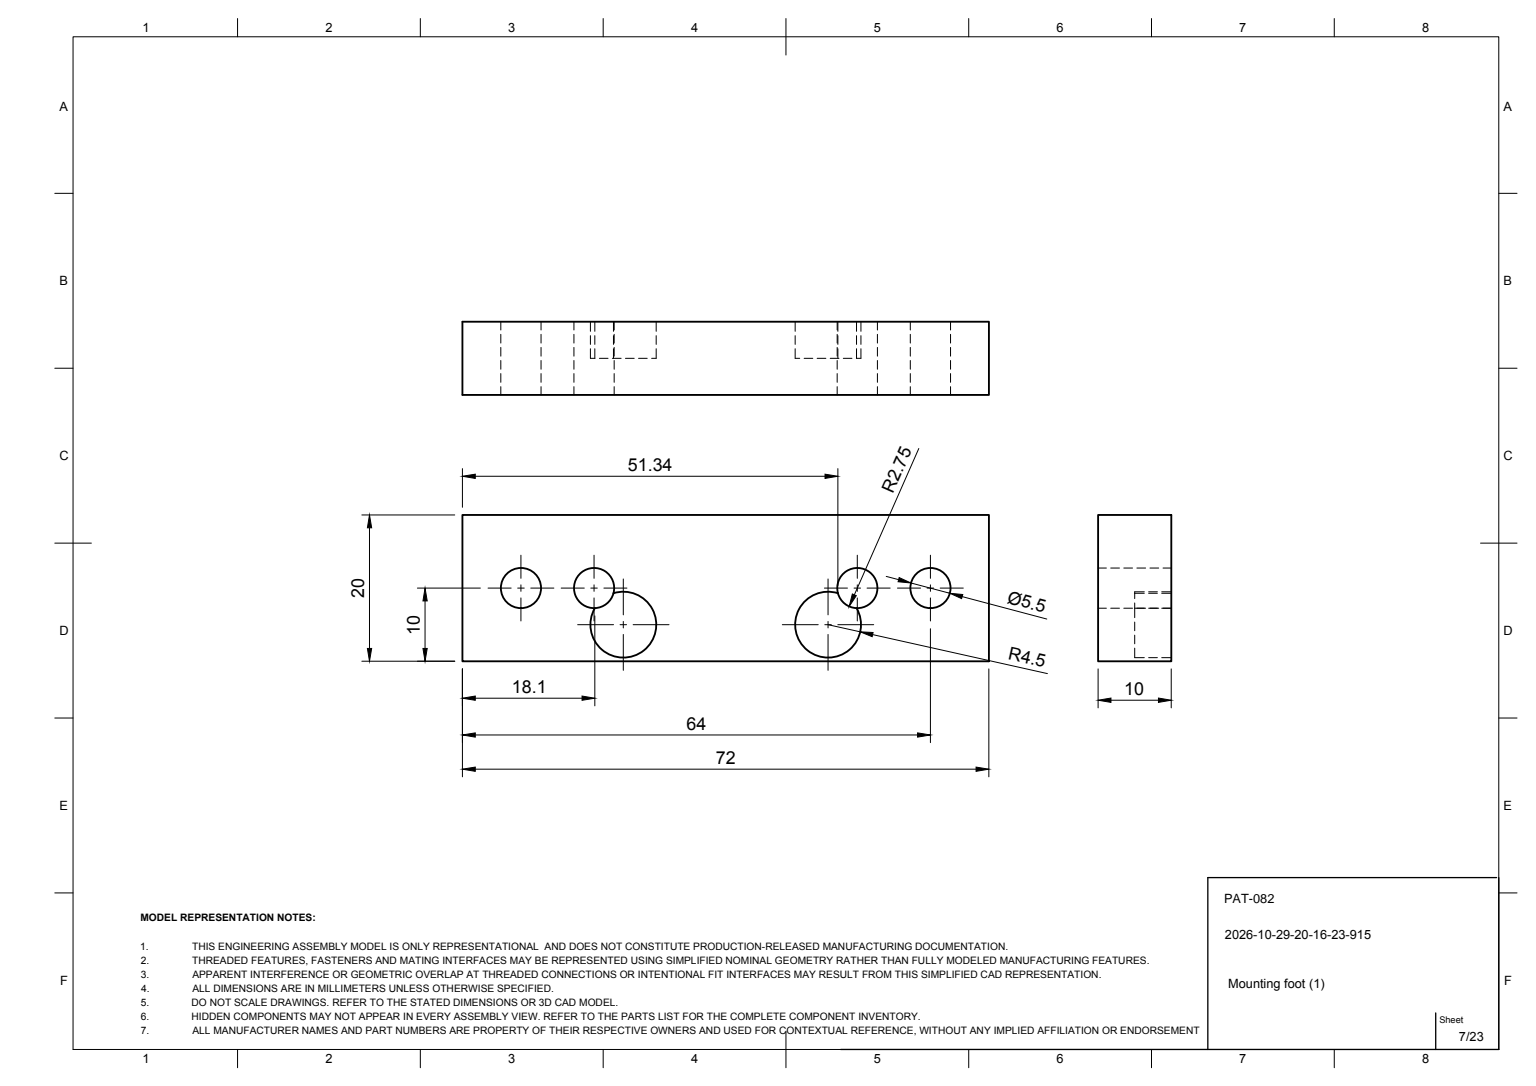
ISO-10303-21;
HEADER;
/* Generated by software containing ST-Developer
 * from STEP Tools, Inc. (www.steptools.com) 
 */

FILE_DESCRIPTION(
/* description */ ('PAT-082'),
/* implementation_level */ '2;1');

FILE_NAME(
/* name */ 'Mounting foot (1).step',
/* time_stamp */ '2026-10-29T20:16:13-07:00',
/* author */ (''),
/* organization */ (''),
/* preprocessor_version */ 'ST-DEVELOPER v20.2',
/* originating_system */ 'Autodesk Translation Framework v15.17.0.0',
/* authorisation */ '');

FILE_SCHEMA (('AUTOMOTIVE_DESIGN { 1 0 10303 214 3 1 1 }'));
ENDSEC;

DATA;
#10=MECHANICAL_DESIGN_GEOMETRIC_PRESENTATION_REPRESENTATION('',(#245),#8266);
#201=SHAPE_REPRESENTATION_RELATIONSHIP('SRR','None',#8363,#223);
#223=ADVANCED_BREP_SHAPE_REPRESENTATION('',(#267),#8247);
#245=STYLED_ITEM('',(#8530),#267);
#267=MANIFOLD_SOLID_BREP('Body1',#4585);
#302=FACE_BOUND('',#919,.T.);
#303=FACE_BOUND('',#920,.T.);
#304=FACE_BOUND('',#921,.T.);
#305=FACE_BOUND('',#922,.T.);
#306=FACE_BOUND('',#924,.T.);
#307=FACE_BOUND('',#925,.T.);
#308=FACE_BOUND('',#926,.T.);
#309=FACE_BOUND('',#927,.T.);
#435=PLANE('',#4931);
#436=PLANE('',#4936);
#437=PLANE('',#4955);
#438=PLANE('',#4956);
#439=PLANE('',#4957);
#440=PLANE('',#4958);
#441=PLANE('',#4959);
#442=PLANE('',#4960);
#616=FACE_OUTER_BOUND('',#906,.T.);
#617=FACE_OUTER_BOUND('',#907,.T.);
#618=FACE_OUTER_BOUND('',#908,.T.);
#619=FACE_OUTER_BOUND('',#909,.T.);
#620=FACE_OUTER_BOUND('',#910,.T.);
#621=FACE_OUTER_BOUND('',#911,.T.);
#622=FACE_OUTER_BOUND('',#912,.T.);
#623=FACE_OUTER_BOUND('',#913,.T.);
#624=FACE_OUTER_BOUND('',#914,.T.);
#625=FACE_OUTER_BOUND('',#915,.T.);
#626=FACE_OUTER_BOUND('',#916,.T.);
#627=FACE_OUTER_BOUND('',#917,.T.);
#628=FACE_OUTER_BOUND('',#918,.T.);
#629=FACE_OUTER_BOUND('',#923,.T.);
#906=EDGE_LOOP('',(#3278,#3279));
#907=EDGE_LOOP('',(#3280,#3281,#3282,#3283));
#908=EDGE_LOOP('',(#3284,#3285));
#909=EDGE_LOOP('',(#3286,#3287,#3288,#3289));
#910=EDGE_LOOP('',(#3290,#3291,#3292,#3293,#3294,#3295,#3296,#3297));
#911=EDGE_LOOP('',(#3298,#3299,#3300,#3301,#3302,#3303,#3304,#3305));
#912=EDGE_LOOP('',(#3306,#3307,#3308,#3309));
#913=EDGE_LOOP('',(#3310,#3311,#3312,#3313));
#914=EDGE_LOOP('',(#3314,#3315,#3316,#3317));
#915=EDGE_LOOP('',(#3318,#3319,#3320,#3321));
#916=EDGE_LOOP('',(#3322,#3323,#3324,#3325));
#917=EDGE_LOOP('',(#3326,#3327,#3328,#3329));
#918=EDGE_LOOP('',(#3330,#3331,#3332,#3333));
#919=EDGE_LOOP('',(#3334,#3335,#3336));
#920=EDGE_LOOP('',(#3337,#3338,#3339));
#921=EDGE_LOOP('',(#3340));
#922=EDGE_LOOP('',(#3341));
#923=EDGE_LOOP('',(#3342,#3343,#3344,#3345));
#924=EDGE_LOOP('',(#3346));
#925=EDGE_LOOP('',(#3347));
#926=EDGE_LOOP('',(#3348));
#927=EDGE_LOOP('',(#3349));
#1299=LINE('',#7020,#1654);
#1300=LINE('',#7023,#1655);
#1301=LINE('',#7031,#1656);
#1302=LINE('',#7034,#1657);
#1303=LINE('',#7039,#1658);
#1304=LINE('',#7046,#1659);
#1305=LINE('',#7053,#1660);
#1306=LINE('',#7059,#1661);
#1307=LINE('',#7064,#1662);
#1308=LINE('',#7066,#1663);
#1309=LINE('',#7068,#1664);
#1310=LINE('',#7069,#1665);
#1311=LINE('',#7072,#1666);
#1312=LINE('',#7074,#1667);
#1313=LINE('',#7075,#1668);
#1314=LINE('',#7078,#1669);
#1315=LINE('',#7080,#1670);
#1316=LINE('',#7081,#1671);
#1317=LINE('',#7083,#1672);
#1318=LINE('',#7084,#1673);
#1654=VECTOR('',#5618,1.);
#1655=VECTOR('',#5621,1.);
#1656=VECTOR('',#5630,1.);
#1657=VECTOR('',#5633,1.);
#1658=VECTOR('',#5638,0.275);
#1659=VECTOR('',#5647,0.275);
#1660=VECTOR('',#5656,0.275);
#1661=VECTOR('',#5663,0.275);
#1662=VECTOR('',#5668,1.);
#1663=VECTOR('',#5669,1.);
#1664=VECTOR('',#5670,1.);
#1665=VECTOR('',#5671,1.);
#1666=VECTOR('',#5674,1.);
#1667=VECTOR('',#5675,1.);
#1668=VECTOR('',#5676,1.);
#1669=VECTOR('',#5679,1.);
#1670=VECTOR('',#5680,1.);
#1671=VECTOR('',#5681,1.);
#1672=VECTOR('',#5684,1.);
#1673=VECTOR('',#5685,1.);
#1977=CIRCLE('',#4932,0.275);
#1978=CIRCLE('',#4933,0.45);
#1979=CIRCLE('',#4935,0.45);
#1980=CIRCLE('',#4937,0.275);
#1981=CIRCLE('',#4938,0.45);
#1982=CIRCLE('',#4940,0.45);
#1983=CIRCLE('',#4942,0.275);
#1984=CIRCLE('',#4943,0.275);
#1985=CIRCLE('',#4944,0.275);
#1986=CIRCLE('',#4946,0.275);
#1987=CIRCLE('',#4947,0.275);
#1988=CIRCLE('',#4948,0.275);
#1989=CIRCLE('',#4950,0.275);
#1990=CIRCLE('',#4951,0.275);
#1991=CIRCLE('',#4953,0.275);
#1992=CIRCLE('',#4954,0.275);
#2209=VERTEX_POINT('',#7014);
#2210=VERTEX_POINT('',#7015);
#2211=VERTEX_POINT('',#7019);
#2212=VERTEX_POINT('',#7021);
#2213=VERTEX_POINT('',#7025);
#2214=VERTEX_POINT('',#7026);
#2215=VERTEX_POINT('',#7030);
#2216=VERTEX_POINT('',#7032);
#2217=VERTEX_POINT('',#7036);
#2218=VERTEX_POINT('',#7038);
#2219=VERTEX_POINT('',#7043);
#2220=VERTEX_POINT('',#7045);
#2221=VERTEX_POINT('',#7050);
#2222=VERTEX_POINT('',#7052);
#2223=VERTEX_POINT('',#7056);
#2224=VERTEX_POINT('',#7058);
#2225=VERTEX_POINT('',#7062);
#2226=VERTEX_POINT('',#7063);
#2227=VERTEX_POINT('',#7065);
#2228=VERTEX_POINT('',#7067);
#2229=VERTEX_POINT('',#7071);
#2230=VERTEX_POINT('',#7073);
#2231=VERTEX_POINT('',#7077);
#2232=VERTEX_POINT('',#7079);
#2615=EDGE_CURVE('',#2209,#2210,#1977,.T.);
#2616=EDGE_CURVE('',#2209,#2210,#1978,.T.);
#2617=EDGE_CURVE('',#2211,#2209,#1299,.T.);
#2618=EDGE_CURVE('',#2212,#2211,#1979,.T.);
#2619=EDGE_CURVE('',#2210,#2212,#1300,.T.);
#2620=EDGE_CURVE('',#2213,#2214,#1980,.T.);
#2621=EDGE_CURVE('',#2213,#2214,#1981,.T.);
#2622=EDGE_CURVE('',#2215,#2213,#1301,.T.);
#2623=EDGE_CURVE('',#2216,#2215,#1982,.T.);
#2624=EDGE_CURVE('',#2214,#2216,#1302,.T.);
#2625=EDGE_CURVE('',#2217,#2217,#1983,.T.);
#2626=EDGE_CURVE('',#2217,#2218,#1303,.T.);
#2627=EDGE_CURVE('',#2211,#2218,#1984,.T.);
#2628=EDGE_CURVE('',#2218,#2212,#1985,.T.);
#2629=EDGE_CURVE('',#2219,#2219,#1986,.T.);
#2630=EDGE_CURVE('',#2219,#2220,#1304,.T.);
#2631=EDGE_CURVE('',#2215,#2220,#1987,.T.);
#2632=EDGE_CURVE('',#2220,#2216,#1988,.T.);
#2633=EDGE_CURVE('',#2221,#2221,#1989,.T.);
#2634=EDGE_CURVE('',#2221,#2222,#1305,.T.);
#2635=EDGE_CURVE('',#2222,#2222,#1990,.T.);
#2636=EDGE_CURVE('',#2223,#2223,#1991,.T.);
#2637=EDGE_CURVE('',#2223,#2224,#1306,.T.);
#2638=EDGE_CURVE('',#2224,#2224,#1992,.T.);
#2639=EDGE_CURVE('',#2225,#2226,#1307,.T.);
#2640=EDGE_CURVE('',#2226,#2227,#1308,.T.);
#2641=EDGE_CURVE('',#2228,#2227,#1309,.T.);
#2642=EDGE_CURVE('',#2225,#2228,#1310,.T.);
#2643=EDGE_CURVE('',#2229,#2225,#1311,.T.);
#2644=EDGE_CURVE('',#2230,#2228,#1312,.T.);
#2645=EDGE_CURVE('',#2229,#2230,#1313,.T.);
#2646=EDGE_CURVE('',#2231,#2229,#1314,.T.);
#2647=EDGE_CURVE('',#2232,#2230,#1315,.T.);
#2648=EDGE_CURVE('',#2231,#2232,#1316,.T.);
#2649=EDGE_CURVE('',#2226,#2231,#1317,.T.);
#2650=EDGE_CURVE('',#2227,#2232,#1318,.T.);
#3278=ORIENTED_EDGE('',*,*,#2615,.F.);
#3279=ORIENTED_EDGE('',*,*,#2616,.T.);
#3280=ORIENTED_EDGE('',*,*,#2617,.F.);
#3281=ORIENTED_EDGE('',*,*,#2618,.F.);
#3282=ORIENTED_EDGE('',*,*,#2619,.F.);
#3283=ORIENTED_EDGE('',*,*,#2616,.F.);
#3284=ORIENTED_EDGE('',*,*,#2620,.F.);
#3285=ORIENTED_EDGE('',*,*,#2621,.T.);
#3286=ORIENTED_EDGE('',*,*,#2622,.F.);
#3287=ORIENTED_EDGE('',*,*,#2623,.F.);
#3288=ORIENTED_EDGE('',*,*,#2624,.F.);
#3289=ORIENTED_EDGE('',*,*,#2621,.F.);
#3290=ORIENTED_EDGE('',*,*,#2625,.F.);
#3291=ORIENTED_EDGE('',*,*,#2626,.T.);
#3292=ORIENTED_EDGE('',*,*,#2627,.F.);
#3293=ORIENTED_EDGE('',*,*,#2617,.T.);
#3294=ORIENTED_EDGE('',*,*,#2615,.T.);
#3295=ORIENTED_EDGE('',*,*,#2619,.T.);
#3296=ORIENTED_EDGE('',*,*,#2628,.F.);
#3297=ORIENTED_EDGE('',*,*,#2626,.F.);
#3298=ORIENTED_EDGE('',*,*,#2629,.F.);
#3299=ORIENTED_EDGE('',*,*,#2630,.T.);
#3300=ORIENTED_EDGE('',*,*,#2631,.F.);
#3301=ORIENTED_EDGE('',*,*,#2622,.T.);
#3302=ORIENTED_EDGE('',*,*,#2620,.T.);
#3303=ORIENTED_EDGE('',*,*,#2624,.T.);
#3304=ORIENTED_EDGE('',*,*,#2632,.F.);
#3305=ORIENTED_EDGE('',*,*,#2630,.F.);
#3306=ORIENTED_EDGE('',*,*,#2633,.F.);
#3307=ORIENTED_EDGE('',*,*,#2634,.T.);
#3308=ORIENTED_EDGE('',*,*,#2635,.F.);
#3309=ORIENTED_EDGE('',*,*,#2634,.F.);
#3310=ORIENTED_EDGE('',*,*,#2636,.F.);
#3311=ORIENTED_EDGE('',*,*,#2637,.T.);
#3312=ORIENTED_EDGE('',*,*,#2638,.F.);
#3313=ORIENTED_EDGE('',*,*,#2637,.F.);
#3314=ORIENTED_EDGE('',*,*,#2639,.T.);
#3315=ORIENTED_EDGE('',*,*,#2640,.T.);
#3316=ORIENTED_EDGE('',*,*,#2641,.F.);
#3317=ORIENTED_EDGE('',*,*,#2642,.F.);
#3318=ORIENTED_EDGE('',*,*,#2643,.T.);
#3319=ORIENTED_EDGE('',*,*,#2642,.T.);
#3320=ORIENTED_EDGE('',*,*,#2644,.F.);
#3321=ORIENTED_EDGE('',*,*,#2645,.F.);
#3322=ORIENTED_EDGE('',*,*,#2646,.T.);
#3323=ORIENTED_EDGE('',*,*,#2645,.T.);
#3324=ORIENTED_EDGE('',*,*,#2647,.F.);
#3325=ORIENTED_EDGE('',*,*,#2648,.F.);
#3326=ORIENTED_EDGE('',*,*,#2649,.T.);
#3327=ORIENTED_EDGE('',*,*,#2648,.T.);
#3328=ORIENTED_EDGE('',*,*,#2650,.F.);
#3329=ORIENTED_EDGE('',*,*,#2640,.F.);
#3330=ORIENTED_EDGE('',*,*,#2650,.T.);
#3331=ORIENTED_EDGE('',*,*,#2647,.T.);
#3332=ORIENTED_EDGE('',*,*,#2644,.T.);
#3333=ORIENTED_EDGE('',*,*,#2641,.T.);
#3334=ORIENTED_EDGE('',*,*,#2618,.T.);
#3335=ORIENTED_EDGE('',*,*,#2627,.T.);
#3336=ORIENTED_EDGE('',*,*,#2628,.T.);
#3337=ORIENTED_EDGE('',*,*,#2623,.T.);
#3338=ORIENTED_EDGE('',*,*,#2631,.T.);
#3339=ORIENTED_EDGE('',*,*,#2632,.T.);
#3340=ORIENTED_EDGE('',*,*,#2635,.T.);
#3341=ORIENTED_EDGE('',*,*,#2638,.T.);
#3342=ORIENTED_EDGE('',*,*,#2649,.F.);
#3343=ORIENTED_EDGE('',*,*,#2639,.F.);
#3344=ORIENTED_EDGE('',*,*,#2643,.F.);
#3345=ORIENTED_EDGE('',*,*,#2646,.F.);
#3346=ORIENTED_EDGE('',*,*,#2625,.T.);
#3347=ORIENTED_EDGE('',*,*,#2633,.T.);
#3348=ORIENTED_EDGE('',*,*,#2636,.T.);
#3349=ORIENTED_EDGE('',*,*,#2629,.T.);
#4234=CYLINDRICAL_SURFACE('',#4934,0.45);
#4235=CYLINDRICAL_SURFACE('',#4939,0.45);
#4236=CYLINDRICAL_SURFACE('',#4941,0.275);
#4237=CYLINDRICAL_SURFACE('',#4945,0.275);
#4238=CYLINDRICAL_SURFACE('',#4949,0.275);
#4239=CYLINDRICAL_SURFACE('',#4952,0.275);
#4355=ADVANCED_FACE('',(#616),#435,.T.);
#4356=ADVANCED_FACE('',(#617),#4234,.F.);
#4357=ADVANCED_FACE('',(#618),#436,.T.);
#4358=ADVANCED_FACE('',(#619),#4235,.F.);
#4359=ADVANCED_FACE('',(#620),#4236,.F.);
#4360=ADVANCED_FACE('',(#621),#4237,.F.);
#4361=ADVANCED_FACE('',(#622),#4238,.F.);
#4362=ADVANCED_FACE('',(#623),#4239,.F.);
#4363=ADVANCED_FACE('',(#624),#437,.T.);
#4364=ADVANCED_FACE('',(#625),#438,.T.);
#4365=ADVANCED_FACE('',(#626),#439,.T.);
#4366=ADVANCED_FACE('',(#627),#440,.T.);
#4367=ADVANCED_FACE('',(#628,#302,#303,#304,#305),#441,.T.);
#4368=ADVANCED_FACE('',(#629,#306,#307,#308,#309),#442,.F.);
#4585=CLOSED_SHELL('',(#4355,#4356,#4357,#4358,#4359,#4360,#4361,#4362,
#4363,#4364,#4365,#4366,#4367,#4368));
#4930=AXIS2_PLACEMENT_3D('',#7012,#5608,#5609);
#4931=AXIS2_PLACEMENT_3D('',#7013,#5610,#5611);
#4932=AXIS2_PLACEMENT_3D('',#7016,#5612,#5613);
#4933=AXIS2_PLACEMENT_3D('',#7017,#5614,#5615);
#4934=AXIS2_PLACEMENT_3D('',#7018,#5616,#5617);
#4935=AXIS2_PLACEMENT_3D('',#7022,#5619,#5620);
#4936=AXIS2_PLACEMENT_3D('',#7024,#5622,#5623);
#4937=AXIS2_PLACEMENT_3D('',#7027,#5624,#5625);
#4938=AXIS2_PLACEMENT_3D('',#7028,#5626,#5627);
#4939=AXIS2_PLACEMENT_3D('',#7029,#5628,#5629);
#4940=AXIS2_PLACEMENT_3D('',#7033,#5631,#5632);
#4941=AXIS2_PLACEMENT_3D('',#7035,#5634,#5635);
#4942=AXIS2_PLACEMENT_3D('',#7037,#5636,#5637);
#4943=AXIS2_PLACEMENT_3D('',#7040,#5639,#5640);
#4944=AXIS2_PLACEMENT_3D('',#7041,#5641,#5642);
#4945=AXIS2_PLACEMENT_3D('',#7042,#5643,#5644);
#4946=AXIS2_PLACEMENT_3D('',#7044,#5645,#5646);
#4947=AXIS2_PLACEMENT_3D('',#7047,#5648,#5649);
#4948=AXIS2_PLACEMENT_3D('',#7048,#5650,#5651);
#4949=AXIS2_PLACEMENT_3D('',#7049,#5652,#5653);
#4950=AXIS2_PLACEMENT_3D('',#7051,#5654,#5655);
#4951=AXIS2_PLACEMENT_3D('',#7054,#5657,#5658);
#4952=AXIS2_PLACEMENT_3D('',#7055,#5659,#5660);
#4953=AXIS2_PLACEMENT_3D('',#7057,#5661,#5662);
#4954=AXIS2_PLACEMENT_3D('',#7060,#5664,#5665);
#4955=AXIS2_PLACEMENT_3D('',#7061,#5666,#5667);
#4956=AXIS2_PLACEMENT_3D('',#7070,#5672,#5673);
#4957=AXIS2_PLACEMENT_3D('',#7076,#5677,#5678);
#4958=AXIS2_PLACEMENT_3D('',#7082,#5682,#5683);
#4959=AXIS2_PLACEMENT_3D('',#7085,#5686,#5687);
#4960=AXIS2_PLACEMENT_3D('',#7086,#5688,#5689);
#5608=DIRECTION('axis',(0.,0.,1.));
#5609=DIRECTION('refdir',(1.,0.,0.));
#5610=DIRECTION('center_axis',(0.,0.,1.));
#5611=DIRECTION('ref_axis',(1.,0.,0.));
#5612=DIRECTION('center_axis',(0.,0.,1.));
#5613=DIRECTION('ref_axis',(1.,0.,0.));
#5614=DIRECTION('center_axis',(0.,0.,1.));
#5615=DIRECTION('ref_axis',(1.,0.,0.));
#5616=DIRECTION('center_axis',(0.,0.,1.));
#5617=DIRECTION('ref_axis',(-0.78086880944303,0.624695047554425,0.));
#5618=DIRECTION('',(0.,0.,-1.));
#5619=DIRECTION('center_axis',(0.,0.,-1.));
#5620=DIRECTION('ref_axis',(1.,0.,0.));
#5621=DIRECTION('',(0.,0.,1.));
#5622=DIRECTION('center_axis',(0.,0.,1.));
#5623=DIRECTION('ref_axis',(1.,0.,0.));
#5624=DIRECTION('center_axis',(0.,0.,1.));
#5625=DIRECTION('ref_axis',(1.,0.,0.));
#5626=DIRECTION('center_axis',(0.,0.,1.));
#5627=DIRECTION('ref_axis',(1.,0.,0.));
#5628=DIRECTION('center_axis',(0.,0.,1.));
#5629=DIRECTION('ref_axis',(-0.78086880944303,-0.624695047554425,0.));
#5630=DIRECTION('',(0.,0.,-1.));
#5631=DIRECTION('center_axis',(0.,0.,-1.));
#5632=DIRECTION('ref_axis',(1.,0.,0.));
#5633=DIRECTION('',(0.,0.,1.));
#5634=DIRECTION('center_axis',(0.,0.,1.));
#5635=DIRECTION('ref_axis',(1.,0.,0.));
#5636=DIRECTION('center_axis',(0.,0.,1.));
#5637=DIRECTION('ref_axis',(1.,0.,0.));
#5638=DIRECTION('',(0.,0.,1.));
#5639=DIRECTION('center_axis',(0.,0.,-1.));
#5640=DIRECTION('ref_axis',(1.,0.,0.));
#5641=DIRECTION('center_axis',(0.,0.,-1.));
#5642=DIRECTION('ref_axis',(1.,0.,0.));
#5643=DIRECTION('center_axis',(0.,0.,1.));
#5644=DIRECTION('ref_axis',(1.,0.,0.));
#5645=DIRECTION('center_axis',(0.,0.,1.));
#5646=DIRECTION('ref_axis',(1.,0.,0.));
#5647=DIRECTION('',(0.,0.,1.));
#5648=DIRECTION('center_axis',(0.,0.,-1.));
#5649=DIRECTION('ref_axis',(1.,0.,0.));
#5650=DIRECTION('center_axis',(0.,0.,-1.));
#5651=DIRECTION('ref_axis',(1.,0.,0.));
#5652=DIRECTION('center_axis',(0.,0.,1.));
#5653=DIRECTION('ref_axis',(1.,0.,0.));
#5654=DIRECTION('center_axis',(0.,0.,1.));
#5655=DIRECTION('ref_axis',(1.,0.,0.));
#5656=DIRECTION('',(0.,0.,1.));
#5657=DIRECTION('center_axis',(0.,0.,-1.));
#5658=DIRECTION('ref_axis',(1.,0.,0.));
#5659=DIRECTION('center_axis',(0.,0.,1.));
#5660=DIRECTION('ref_axis',(1.,0.,0.));
#5661=DIRECTION('center_axis',(0.,0.,1.));
#5662=DIRECTION('ref_axis',(1.,0.,0.));
#5663=DIRECTION('',(0.,0.,1.));
#5664=DIRECTION('center_axis',(0.,0.,-1.));
#5665=DIRECTION('ref_axis',(1.,0.,0.));
#5666=DIRECTION('center_axis',(0.,1.,0.));
#5667=DIRECTION('ref_axis',(-1.,0.,0.));
#5668=DIRECTION('',(-1.,0.,0.));
#5669=DIRECTION('',(0.,0.,1.));
#5670=DIRECTION('',(-1.,0.,0.));
#5671=DIRECTION('',(0.,0.,1.));
#5672=DIRECTION('center_axis',(1.,0.,0.));
#5673=DIRECTION('ref_axis',(0.,1.,0.));
#5674=DIRECTION('',(0.,1.,0.));
#5675=DIRECTION('',(0.,1.,0.));
#5676=DIRECTION('',(0.,0.,1.));
#5677=DIRECTION('center_axis',(0.,-1.,0.));
#5678=DIRECTION('ref_axis',(1.,0.,0.));
#5679=DIRECTION('',(1.,0.,0.));
#5680=DIRECTION('',(1.,0.,0.));
#5681=DIRECTION('',(0.,0.,1.));
#5682=DIRECTION('center_axis',(-1.,0.,0.));
#5683=DIRECTION('ref_axis',(0.,-1.,0.));
#5684=DIRECTION('',(0.,-1.,0.));
#5685=DIRECTION('',(0.,-1.,0.));
#5686=DIRECTION('center_axis',(0.,0.,1.));
#5687=DIRECTION('ref_axis',(1.,0.,0.));
#5688=DIRECTION('center_axis',(0.,0.,1.));
#5689=DIRECTION('ref_axis',(1.,0.,0.));
#7012=CARTESIAN_POINT('',(0.,0.,0.));
#7013=CARTESIAN_POINT('Origin',(4.5,-1.4,0.9));
#7014=CARTESIAN_POINT('',(4.92952879918449,-1.53418275101939,0.9));
#7015=CARTESIAN_POINT('',(4.72519681057161,-1.78959773678549,0.9));
#7016=CARTESIAN_POINT('Origin',(5.,-1.8,0.9));
#7017=CARTESIAN_POINT('Origin',(4.5,-1.4,0.9));
#7018=CARTESIAN_POINT('Origin',(4.5,-1.4,0.9));
#7019=CARTESIAN_POINT('',(4.92952879918449,-1.53418275101939,1.4));
#7020=CARTESIAN_POINT('',(4.92952879918449,-1.53418275101939,0.9));
#7021=CARTESIAN_POINT('',(4.72519681057161,-1.78959773678549,1.4));
#7022=CARTESIAN_POINT('Origin',(4.5,-1.4,1.4));
#7023=CARTESIAN_POINT('',(4.72519681057161,-1.78959773678549,0.9));
#7024=CARTESIAN_POINT('Origin',(4.5,1.4,0.9));
#7025=CARTESIAN_POINT('',(4.72519681057161,1.78959773678549,0.9));
#7026=CARTESIAN_POINT('',(4.92952879918449,1.53418275101939,0.9));
#7027=CARTESIAN_POINT('Origin',(5.,1.8,0.9));
#7028=CARTESIAN_POINT('Origin',(4.5,1.4,0.9));
#7029=CARTESIAN_POINT('Origin',(4.5,1.4,0.9));
#7030=CARTESIAN_POINT('',(4.72519681057161,1.78959773678549,1.4));
#7031=CARTESIAN_POINT('',(4.72519681057161,1.78959773678549,0.9));
#7032=CARTESIAN_POINT('',(4.92952879918449,1.53418275101939,1.4));
#7033=CARTESIAN_POINT('Origin',(4.5,1.4,1.4));
#7034=CARTESIAN_POINT('',(4.92952879918449,1.53418275101939,0.9));
#7035=CARTESIAN_POINT('Origin',(5.,-1.8,0.3));
#7036=CARTESIAN_POINT('',(4.725,-1.8,0.4));
#7037=CARTESIAN_POINT('Origin',(5.,-1.8,0.4));
#7038=CARTESIAN_POINT('',(4.725,-1.8,1.4));
#7039=CARTESIAN_POINT('',(4.725,-1.8,0.3));
#7040=CARTESIAN_POINT('Origin',(5.,-1.8,1.4));
#7041=CARTESIAN_POINT('Origin',(5.,-1.8,1.4));
#7042=CARTESIAN_POINT('Origin',(5.,1.8,0.3));
#7043=CARTESIAN_POINT('',(4.725,1.8,0.4));
#7044=CARTESIAN_POINT('Origin',(5.,1.8,0.4));
#7045=CARTESIAN_POINT('',(4.725,1.8,1.4));
#7046=CARTESIAN_POINT('',(4.725,1.8,0.3));
#7047=CARTESIAN_POINT('Origin',(5.,1.8,1.4));
#7048=CARTESIAN_POINT('Origin',(5.,1.8,1.4));
#7049=CARTESIAN_POINT('Origin',(5.,2.8,0.3));
#7050=CARTESIAN_POINT('',(4.725,2.8,0.4));
#7051=CARTESIAN_POINT('Origin',(5.,2.8,0.4));
#7052=CARTESIAN_POINT('',(4.725,2.8,1.4));
#7053=CARTESIAN_POINT('',(4.725,2.8,0.3));
#7054=CARTESIAN_POINT('Origin',(5.,2.8,1.4));
#7055=CARTESIAN_POINT('Origin',(5.,-2.8,0.3));
#7056=CARTESIAN_POINT('',(4.725,-2.8,0.4));
#7057=CARTESIAN_POINT('Origin',(5.,-2.8,0.4));
#7058=CARTESIAN_POINT('',(4.725,-2.8,1.4));
#7059=CARTESIAN_POINT('',(4.725,-2.8,0.3));
#7060=CARTESIAN_POINT('Origin',(5.,-2.8,1.4));
#7061=CARTESIAN_POINT('Origin',(6.,3.6,0.4));
#7062=CARTESIAN_POINT('',(6.,3.6,0.4));
#7063=CARTESIAN_POINT('',(4.,3.6,0.4));
#7064=CARTESIAN_POINT('',(6.,3.6,0.4));
#7065=CARTESIAN_POINT('',(4.,3.6,1.4));
#7066=CARTESIAN_POINT('',(4.,3.6,0.4));
#7067=CARTESIAN_POINT('',(6.,3.6,1.4));
#7068=CARTESIAN_POINT('',(6.,3.6,1.4));
#7069=CARTESIAN_POINT('',(6.,3.6,0.4));
#7070=CARTESIAN_POINT('Origin',(6.,-3.6,0.4));
#7071=CARTESIAN_POINT('',(6.,-3.6,0.4));
#7072=CARTESIAN_POINT('',(6.,-3.6,0.4));
#7073=CARTESIAN_POINT('',(6.,-3.6,1.4));
#7074=CARTESIAN_POINT('',(6.,-3.6,1.4));
#7075=CARTESIAN_POINT('',(6.,-3.6,0.4));
#7076=CARTESIAN_POINT('Origin',(4.,-3.6,0.4));
#7077=CARTESIAN_POINT('',(4.,-3.6,0.4));
#7078=CARTESIAN_POINT('',(4.,-3.6,0.4));
#7079=CARTESIAN_POINT('',(4.,-3.6,1.4));
#7080=CARTESIAN_POINT('',(4.,-3.6,1.4));
#7081=CARTESIAN_POINT('',(4.,-3.6,0.4));
#7082=CARTESIAN_POINT('Origin',(4.,3.6,0.4));
#7083=CARTESIAN_POINT('',(4.,3.6,0.4));
#7084=CARTESIAN_POINT('',(4.,3.6,1.4));
#7085=CARTESIAN_POINT('Origin',(5.,0.,1.4));
#7086=CARTESIAN_POINT('Origin',(5.,0.,0.4));
#8222=UNCERTAINTY_MEASURE_WITH_UNIT(LENGTH_MEASURE(0.001),#8267,
'DISTANCE_ACCURACY_VALUE',
'Maximum model space distance between geometric entities at asserted c
onnectivities');
#8241=UNCERTAINTY_MEASURE_WITH_UNIT(LENGTH_MEASURE(0.001),#8267,
'DISTANCE_ACCURACY_VALUE',
'Maximum model space distance between geometric entities at asserted c
onnectivities');
#8247=(
GEOMETRIC_REPRESENTATION_CONTEXT(3)
GLOBAL_UNCERTAINTY_ASSIGNED_CONTEXT((#8222))
GLOBAL_UNIT_ASSIGNED_CONTEXT((#8267,#8269,#8270))
REPRESENTATION_CONTEXT('','3D')
);
#8266=(
GEOMETRIC_REPRESENTATION_CONTEXT(3)
GLOBAL_UNCERTAINTY_ASSIGNED_CONTEXT((#8241))
GLOBAL_UNIT_ASSIGNED_CONTEXT((#8267,#8269,#8270))
REPRESENTATION_CONTEXT('','3D')
);
#8267=(
LENGTH_UNIT()
NAMED_UNIT(*)
SI_UNIT(.CENTI.,.METRE.)
);
#8269=(
NAMED_UNIT(*)
PLANE_ANGLE_UNIT()
SI_UNIT($,.RADIAN.)
);
#8270=(
NAMED_UNIT(*)
SI_UNIT($,.STERADIAN.)
SOLID_ANGLE_UNIT()
);
#8276=SHAPE_DEFINITION_REPRESENTATION(#8300,#8363);
#8300=PRODUCT_DEFINITION_SHAPE('',$,#8388);
#8363=SHAPE_REPRESENTATION('',(#4930),#8247);
#8382=PRODUCT_DEFINITION_CONTEXT('part definition',#8456,'design');
#8388=PRODUCT_DEFINITION('Mounting foot (1)','Mounting foot (1)',
#8412,#8382);
#8412=PRODUCT_DEFINITION_FORMATION('',$,#8463);
#8456=APPLICATION_CONTEXT(
'Core Data for Automotive Mechanical Design Process');
#8457=PRODUCT_CONTEXT('part definition',#8456,'mechanical');
#8463=PRODUCT('Mounting foot (1)','Mounting foot (1)',
'Mounting foot (1)',(#8457));
#8524=COLOUR_RGB('Sky Blue',0.24,0.69,0.87);
#8525=FILL_AREA_STYLE_COLOUR('',#8524);
#8526=FILL_AREA_STYLE('',(#8525));
#8527=SURFACE_STYLE_FILL_AREA(#8526);
#8528=SURFACE_SIDE_STYLE('',(#8527));
#8529=SURFACE_STYLE_USAGE(.BOTH.,#8528);
#8530=PRESENTATION_STYLE_ASSIGNMENT((#8529));
ENDSEC;
END-ISO-10303-21;
